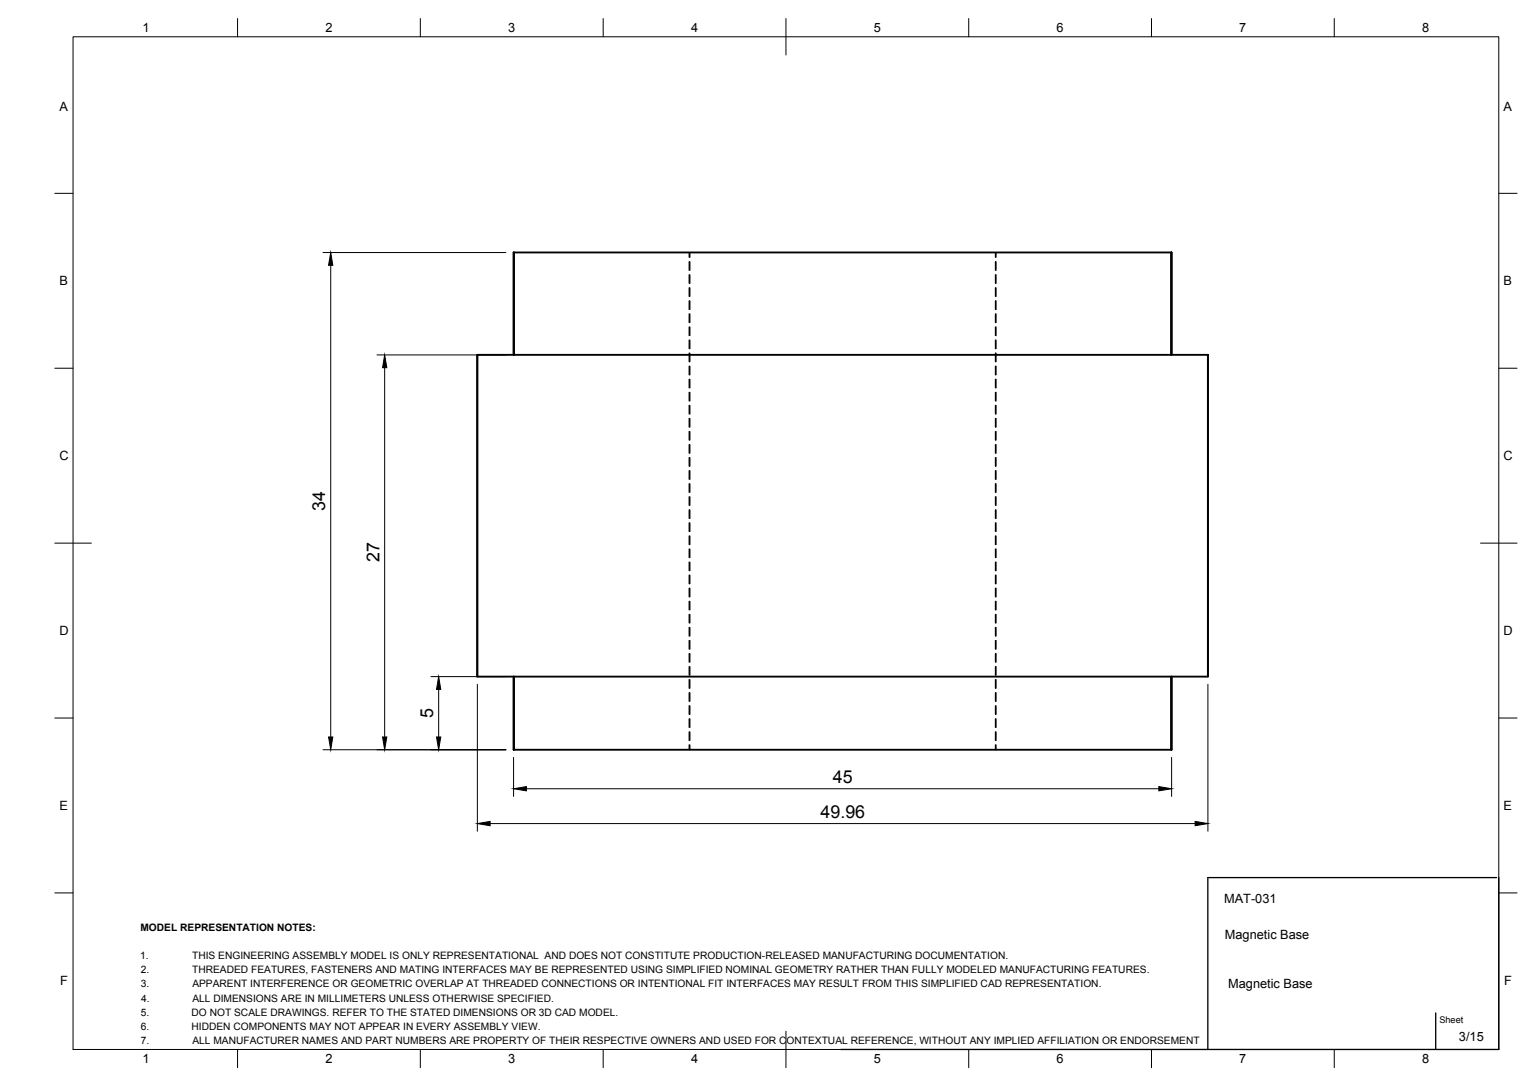
ISO-10303-21;
HEADER;
/* Generated by software containing ST-Developer
 * from STEP Tools, Inc. (www.steptools.com) 
 */

FILE_DESCRIPTION(
/* description */ ('STEP AP214'),
/* implementation_level */ '2;1');

FILE_NAME(
/* name */ 'Magnetic Base.step',
/* time_stamp */ '2026-11-14T06:58:01-08:00',
/* author */ (''),
/* organization */ (''),
/* preprocessor_version */ 'ST-DEVELOPER v20.2',
/* originating_system */ 'Autodesk Translation Framework v15.17.0.0',
/* authorisation */ '');

FILE_SCHEMA (('AUTOMOTIVE_DESIGN { 1 0 10303 214 3 1 1 }'));
ENDSEC;

DATA;
#10=MECHANICAL_DESIGN_GEOMETRIC_PRESENTATION_REPRESENTATION('',(#1140,#1141,#1142,#1143),#38635);
#1112=SHAPE_REPRESENTATION_RELATIONSHIP('SRR','None',#38685,#1126);
#1126=ADVANCED_BREP_SHAPE_REPRESENTATION('',(#1166,#1167,#1168,#1169),#38621);
#1140=STYLED_ITEM('',(#38764),#1166);
#1141=STYLED_ITEM('',(#38764),#1167);
#1142=STYLED_ITEM('',(#38764),#1168);
#1143=STYLED_ITEM('',(#38764),#1169);
#1166=MANIFOLD_SOLID_BREP('Body1',#17606);
#1167=MANIFOLD_SOLID_BREP('Body2',#17607);
#1168=MANIFOLD_SOLID_BREP('Body3',#17608);
#1169=MANIFOLD_SOLID_BREP('Body4',#17609);
#1192=PLANE('',#17795);
#1193=PLANE('',#17796);
#1194=PLANE('',#17797);
#1195=PLANE('',#17800);
#1196=PLANE('',#17803);
#1197=PLANE('',#17804);
#1198=PLANE('',#17816);
#1199=PLANE('',#17817);
#1200=PLANE('',#17818);
#1201=PLANE('',#17819);
#1202=PLANE('',#17821);
#1203=PLANE('',#17824);
#1204=PLANE('',#17825);
#1205=PLANE('',#17826);
#1206=PLANE('',#17827);
#1207=PLANE('',#17828);
#1208=PLANE('',#17831);
#1209=PLANE('',#17835);
#1210=PLANE('',#17838);
#1211=PLANE('',#17841);
#1212=PLANE('',#17842);
#1213=PLANE('',#17843);
#1214=PLANE('',#17844);
#1215=PLANE('',#17847);
#1216=PLANE('',#17851);
#1217=PLANE('',#17854);
#1641=FACE_OUTER_BOUND('',#2647,.T.);
#1642=FACE_OUTER_BOUND('',#2648,.T.);
#1643=FACE_OUTER_BOUND('',#2649,.T.);
#1644=FACE_OUTER_BOUND('',#2650,.T.);
#1645=FACE_OUTER_BOUND('',#2651,.T.);
#1646=FACE_OUTER_BOUND('',#2652,.T.);
#1647=FACE_OUTER_BOUND('',#2653,.T.);
#1648=FACE_OUTER_BOUND('',#2654,.T.);
#1649=FACE_OUTER_BOUND('',#2655,.T.);
#1650=FACE_OUTER_BOUND('',#2656,.T.);
#1651=FACE_OUTER_BOUND('',#2657,.T.);
#1652=FACE_OUTER_BOUND('',#2658,.T.);
#1653=FACE_OUTER_BOUND('',#2659,.T.);
#1654=FACE_OUTER_BOUND('',#2660,.T.);
#1655=FACE_OUTER_BOUND('',#2661,.T.);
#1656=FACE_OUTER_BOUND('',#2662,.T.);
#1657=FACE_OUTER_BOUND('',#2663,.T.);
#1658=FACE_OUTER_BOUND('',#2664,.T.);
#1659=FACE_OUTER_BOUND('',#2665,.T.);
#1660=FACE_OUTER_BOUND('',#2666,.T.);
#1661=FACE_OUTER_BOUND('',#2667,.T.);
#1662=FACE_OUTER_BOUND('',#2668,.T.);
#1663=FACE_OUTER_BOUND('',#2669,.T.);
#1664=FACE_OUTER_BOUND('',#2670,.T.);
#1665=FACE_OUTER_BOUND('',#2671,.T.);
#1666=FACE_OUTER_BOUND('',#2672,.T.);
#1667=FACE_OUTER_BOUND('',#2673,.T.);
#1668=FACE_OUTER_BOUND('',#2674,.T.);
#1669=FACE_OUTER_BOUND('',#2675,.T.);
#1670=FACE_OUTER_BOUND('',#2676,.T.);
#1671=FACE_OUTER_BOUND('',#2677,.T.);
#1672=FACE_OUTER_BOUND('',#2678,.T.);
#1673=FACE_OUTER_BOUND('',#2679,.T.);
#1674=FACE_OUTER_BOUND('',#2680,.T.);
#1675=FACE_OUTER_BOUND('',#2681,.T.);
#1676=FACE_OUTER_BOUND('',#2682,.T.);
#1677=FACE_OUTER_BOUND('',#2683,.T.);
#1678=FACE_OUTER_BOUND('',#2684,.T.);
#1679=FACE_OUTER_BOUND('',#2685,.T.);
#1680=FACE_OUTER_BOUND('',#2686,.T.);
#2647=EDGE_LOOP('',(#10909,#10910,#10911,#10912));
#2648=EDGE_LOOP('',(#10913,#10914,#10915,#10916));
#2649=EDGE_LOOP('',(#10917,#10918,#10919,#10920,#10921,#10922,#10923,#10924));
#2650=EDGE_LOOP('',(#10925,#10926,#10927,#10928,#10929,#10930,#10931,#10932));
#2651=EDGE_LOOP('',(#10933,#10934,#10935,#10936));
#2652=EDGE_LOOP('',(#10937,#10938,#10939,#10940));
#2653=EDGE_LOOP('',(#10941,#10942,#10943,#10944));
#2654=EDGE_LOOP('',(#10945,#10946,#10947,#10948));
#2655=EDGE_LOOP('',(#10949,#10950,#10951,#10952));
#2656=EDGE_LOOP('',(#10953,#10954,#10955,#10956));
#2657=EDGE_LOOP('',(#10957,#10958,#10959,#10960));
#2658=EDGE_LOOP('',(#10961,#10962,#10963,#10964));
#2659=EDGE_LOOP('',(#10965,#10966,#10967,#10968));
#2660=EDGE_LOOP('',(#10969,#10970,#10971,#10972,#10973,#10974,#10975,#10976));
#2661=EDGE_LOOP('',(#10977,#10978,#10979,#10980,#10981,#10982,#10983,#10984));
#2662=EDGE_LOOP('',(#10985,#10986,#10987,#10988));
#2663=EDGE_LOOP('',(#10989,#10990,#10991,#10992));
#2664=EDGE_LOOP('',(#10993,#10994,#10995,#10996));
#2665=EDGE_LOOP('',(#10997,#10998,#10999,#11000));
#2666=EDGE_LOOP('',(#11001,#11002,#11003,#11004));
#2667=EDGE_LOOP('',(#11005,#11006,#11007,#11008));
#2668=EDGE_LOOP('',(#11009,#11010,#11011,#11012,#11013,#11014,#11015,#11016));
#2669=EDGE_LOOP('',(#11017,#11018,#11019,#11020,#11021,#11022,#11023,#11024));
#2670=EDGE_LOOP('',(#11025,#11026,#11027,#11028));
#2671=EDGE_LOOP('',(#11029,#11030,#11031,#11032));
#2672=EDGE_LOOP('',(#11033,#11034,#11035,#11036));
#2673=EDGE_LOOP('',(#11037,#11038,#11039,#11040));
#2674=EDGE_LOOP('',(#11041,#11042,#11043,#11044));
#2675=EDGE_LOOP('',(#11045,#11046,#11047,#11048));
#2676=EDGE_LOOP('',(#11049,#11050,#11051,#11052));
#2677=EDGE_LOOP('',(#11053,#11054,#11055,#11056));
#2678=EDGE_LOOP('',(#11057,#11058,#11059,#11060,#11061,#11062,#11063,#11064));
#2679=EDGE_LOOP('',(#11065,#11066,#11067,#11068,#11069,#11070,#11071,#11072));
#2680=EDGE_LOOP('',(#11073,#11074,#11075,#11076));
#2681=EDGE_LOOP('',(#11077,#11078,#11079,#11080));
#2682=EDGE_LOOP('',(#11081,#11082,#11083,#11084));
#2683=EDGE_LOOP('',(#11085,#11086,#11087,#11088));
#2684=EDGE_LOOP('',(#11089,#11090,#11091,#11092));
#2685=EDGE_LOOP('',(#11093,#11094,#11095,#11096));
#2686=EDGE_LOOP('',(#11097,#11098,#11099,#11100));
#3698=LINE('',#24606,#4642);
#3699=LINE('',#24609,#4643);
#3700=LINE('',#24615,#4644);
#3701=LINE('',#24618,#4645);
#3702=LINE('',#24621,#4646);
#3703=LINE('',#24623,#4647);
#3704=LINE('',#24625,#4648);
#3705=LINE('',#24627,#4649);
#3706=LINE('',#24628,#4650);
#3707=LINE('',#24629,#4651);
#3708=LINE('',#24632,#4652);
#3709=LINE('',#24633,#4653);
#3710=LINE('',#24635,#4654);
#3711=LINE('',#24637,#4655);
#3712=LINE('',#24639,#4656);
#3713=LINE('',#24640,#4657);
#3714=LINE('',#24656,#4658);
#3715=LINE('',#24659,#4659);
#3716=LINE('',#24665,#4660);
#3717=LINE('',#24668,#4661);
#3718=LINE('',#24674,#4662);
#3719=LINE('',#24677,#4663);
#3720=LINE('',#24679,#4664);
#3721=LINE('',#24680,#4665);
#3722=LINE('',#24682,#4666);
#3723=LINE('',#24684,#4667);
#3724=LINE('',#24685,#4668);
#3725=LINE('',#24687,#4669);
#3726=LINE('',#24689,#4670);
#3727=LINE('',#24691,#4671);
#3728=LINE('',#24692,#4672);
#3729=LINE('',#24693,#4673);
#3730=LINE('',#24704,#4674);
#3731=LINE('',#24706,#4675);
#3732=LINE('',#24708,#4676);
#3733=LINE('',#24709,#4677);
#3734=LINE('',#24713,#4678);
#3735=LINE('',#24714,#4679);
#3736=LINE('',#24716,#4680);
#3737=LINE('',#24718,#4681);
#3738=LINE('',#24720,#4682);
#3739=LINE('',#24722,#4683);
#3740=LINE('',#24723,#4684);
#3741=LINE('',#24726,#4685);
#3742=LINE('',#24728,#4686);
#3743=LINE('',#24730,#4687);
#3744=LINE('',#24732,#4688);
#3745=LINE('',#24734,#4689);
#3746=LINE('',#24736,#4690);
#3747=LINE('',#24737,#4691);
#3748=LINE('',#24754,#4692);
#3749=LINE('',#24756,#4693);
#3750=LINE('',#24758,#4694);
#3751=LINE('',#24759,#4695);
#3752=LINE('',#24763,#4696);
#3753=LINE('',#24764,#4697);
#3754=LINE('',#24766,#4698);
#3755=LINE('',#24768,#4699);
#3756=LINE('',#24770,#4700);
#3757=LINE('',#24772,#4701);
#3758=LINE('',#24773,#4702);
#3759=LINE('',#24776,#4703);
#3760=LINE('',#24778,#4704);
#3761=LINE('',#24780,#4705);
#3762=LINE('',#24782,#4706);
#3763=LINE('',#24784,#4707);
#3764=LINE('',#24786,#4708);
#3765=LINE('',#24787,#4709);
#4642=VECTOR('',#19751,1000.);
#4643=VECTOR('',#19754,1000.);
#4644=VECTOR('',#19759,1000.);
#4645=VECTOR('',#19762,1000.);
#4646=VECTOR('',#19765,1000.);
#4647=VECTOR('',#19766,1000.);
#4648=VECTOR('',#19767,1000.);
#4649=VECTOR('',#19768,1000.);
#4650=VECTOR('',#19769,1000.);
#4651=VECTOR('',#19770,1000.);
#4652=VECTOR('',#19773,1000.);
#4653=VECTOR('',#19774,1000.);
#4654=VECTOR('',#19775,1000.);
#4655=VECTOR('',#19776,1000.);
#4656=VECTOR('',#19777,1000.);
#4657=VECTOR('',#19778,1000.);
#4658=VECTOR('',#19803,1000.);
#4659=VECTOR('',#19806,1000.);
#4660=VECTOR('',#19811,1000.);
#4661=VECTOR('',#19814,1000.);
#4662=VECTOR('',#19819,1000.);
#4663=VECTOR('',#19822,1000.);
#4664=VECTOR('',#19825,1000.);
#4665=VECTOR('',#19826,1000.);
#4666=VECTOR('',#19827,1000.);
#4667=VECTOR('',#19828,1000.);
#4668=VECTOR('',#19829,1000.);
#4669=VECTOR('',#19832,1000.);
#4670=VECTOR('',#19833,1000.);
#4671=VECTOR('',#19834,1000.);
#4672=VECTOR('',#19835,1000.);
#4673=VECTOR('',#19836,1000.);
#4674=VECTOR('',#19853,1000.);
#4675=VECTOR('',#19854,1000.);
#4676=VECTOR('',#19855,1000.);
#4677=VECTOR('',#19856,1000.);
#4678=VECTOR('',#19859,1000.);
#4679=VECTOR('',#19860,1000.);
#4680=VECTOR('',#19861,1000.);
#4681=VECTOR('',#19862,1000.);
#4682=VECTOR('',#19863,1000.);
#4683=VECTOR('',#19864,1000.);
#4684=VECTOR('',#19865,1000.);
#4685=VECTOR('',#19868,1000.);
#4686=VECTOR('',#19869,1000.);
#4687=VECTOR('',#19870,1000.);
#4688=VECTOR('',#19871,1000.);
#4689=VECTOR('',#19872,1000.);
#4690=VECTOR('',#19873,1000.);
#4691=VECTOR('',#19874,1000.);
#4692=VECTOR('',#19903,1000.);
#4693=VECTOR('',#19904,1000.);
#4694=VECTOR('',#19905,1000.);
#4695=VECTOR('',#19906,1000.);
#4696=VECTOR('',#19909,1000.);
#4697=VECTOR('',#19910,1000.);
#4698=VECTOR('',#19911,1000.);
#4699=VECTOR('',#19912,1000.);
#4700=VECTOR('',#19913,1000.);
#4701=VECTOR('',#19914,1000.);
#4702=VECTOR('',#19915,1000.);
#4703=VECTOR('',#19918,1000.);
#4704=VECTOR('',#19919,1000.);
#4705=VECTOR('',#19920,1000.);
#4706=VECTOR('',#19921,1000.);
#4707=VECTOR('',#19922,1000.);
#4708=VECTOR('',#19923,1000.);
#4709=VECTOR('',#19924,1000.);
#5586=CIRCLE('',#17790,22.5);
#5587=CIRCLE('',#17791,22.5);
#5588=CIRCLE('',#17793,25.);
#5589=CIRCLE('',#17794,25.);
#5590=CIRCLE('',#17798,22.5);
#5591=CIRCLE('',#17799,10.5);
#5592=CIRCLE('',#17801,10.5);
#5593=CIRCLE('',#17805,22.5);
#5594=CIRCLE('',#17808,22.5);
#5595=CIRCLE('',#17809,22.5);
#5596=CIRCLE('',#17811,10.5);
#5597=CIRCLE('',#17812,10.5);
#5598=CIRCLE('',#17814,25.);
#5599=CIRCLE('',#17815,25.);
#5600=CIRCLE('',#17820,22.5);
#5601=CIRCLE('',#17822,22.5);
#5602=CIRCLE('',#17829,22.5);
#5603=CIRCLE('',#17830,10.5);
#5604=CIRCLE('',#17832,22.5);
#5605=CIRCLE('',#17833,10.5);
#5606=CIRCLE('',#17836,22.5);
#5607=CIRCLE('',#17839,22.5);
#5608=CIRCLE('',#17845,22.5);
#5609=CIRCLE('',#17846,10.5);
#5610=CIRCLE('',#17848,22.5);
#5611=CIRCLE('',#17849,10.5);
#5612=CIRCLE('',#17852,22.5);
#5613=CIRCLE('',#17855,22.5);
#6512=VERTEX_POINT('',#24602);
#6513=VERTEX_POINT('',#24603);
#6514=VERTEX_POINT('',#24605);
#6515=VERTEX_POINT('',#24607);
#6516=VERTEX_POINT('',#24611);
#6517=VERTEX_POINT('',#24612);
#6518=VERTEX_POINT('',#24614);
#6519=VERTEX_POINT('',#24616);
#6520=VERTEX_POINT('',#24620);
#6521=VERTEX_POINT('',#24622);
#6522=VERTEX_POINT('',#24624);
#6523=VERTEX_POINT('',#24626);
#6524=VERTEX_POINT('',#24631);
#6525=VERTEX_POINT('',#24634);
#6526=VERTEX_POINT('',#24636);
#6527=VERTEX_POINT('',#24638);
#6528=VERTEX_POINT('',#24652);
#6529=VERTEX_POINT('',#24653);
#6530=VERTEX_POINT('',#24655);
#6531=VERTEX_POINT('',#24657);
#6532=VERTEX_POINT('',#24661);
#6533=VERTEX_POINT('',#24662);
#6534=VERTEX_POINT('',#24664);
#6535=VERTEX_POINT('',#24666);
#6536=VERTEX_POINT('',#24670);
#6537=VERTEX_POINT('',#24671);
#6538=VERTEX_POINT('',#24673);
#6539=VERTEX_POINT('',#24675);
#6540=VERTEX_POINT('',#24681);
#6541=VERTEX_POINT('',#24683);
#6542=VERTEX_POINT('',#24688);
#6543=VERTEX_POINT('',#24690);
#6544=VERTEX_POINT('',#24702);
#6545=VERTEX_POINT('',#24703);
#6546=VERTEX_POINT('',#24705);
#6547=VERTEX_POINT('',#24707);
#6548=VERTEX_POINT('',#24711);
#6549=VERTEX_POINT('',#24712);
#6550=VERTEX_POINT('',#24715);
#6551=VERTEX_POINT('',#24717);
#6552=VERTEX_POINT('',#24719);
#6553=VERTEX_POINT('',#24721);
#6554=VERTEX_POINT('',#24725);
#6555=VERTEX_POINT('',#24727);
#6556=VERTEX_POINT('',#24729);
#6557=VERTEX_POINT('',#24731);
#6558=VERTEX_POINT('',#24733);
#6559=VERTEX_POINT('',#24735);
#6560=VERTEX_POINT('',#24752);
#6561=VERTEX_POINT('',#24753);
#6562=VERTEX_POINT('',#24755);
#6563=VERTEX_POINT('',#24757);
#6564=VERTEX_POINT('',#24761);
#6565=VERTEX_POINT('',#24762);
#6566=VERTEX_POINT('',#24765);
#6567=VERTEX_POINT('',#24767);
#6568=VERTEX_POINT('',#24769);
#6569=VERTEX_POINT('',#24771);
#6570=VERTEX_POINT('',#24775);
#6571=VERTEX_POINT('',#24777);
#6572=VERTEX_POINT('',#24779);
#6573=VERTEX_POINT('',#24781);
#6574=VERTEX_POINT('',#24783);
#6575=VERTEX_POINT('',#24785);
#8241=EDGE_CURVE('',#6512,#6513,#5586,.T.);
#8242=EDGE_CURVE('',#6513,#6514,#3698,.T.);
#8243=EDGE_CURVE('',#6515,#6514,#5587,.T.);
#8244=EDGE_CURVE('',#6515,#6512,#3699,.T.);
#8245=EDGE_CURVE('',#6516,#6517,#5588,.T.);
#8246=EDGE_CURVE('',#6516,#6518,#3700,.T.);
#8247=EDGE_CURVE('',#6519,#6518,#5589,.T.);
#8248=EDGE_CURVE('',#6519,#6517,#3701,.T.);
#8249=EDGE_CURVE('',#6520,#6516,#3702,.T.);
#8250=EDGE_CURVE('',#6521,#6520,#3703,.T.);
#8251=EDGE_CURVE('',#6522,#6521,#3704,.T.);
#8252=EDGE_CURVE('',#6522,#6523,#3705,.T.);
#8253=EDGE_CURVE('',#6523,#6514,#3706,.T.);
#8254=EDGE_CURVE('',#6518,#6513,#3707,.T.);
#8255=EDGE_CURVE('',#6517,#6524,#3708,.T.);
#8256=EDGE_CURVE('',#6512,#6519,#3709,.T.);
#8257=EDGE_CURVE('',#6515,#6525,#3710,.T.);
#8258=EDGE_CURVE('',#6525,#6526,#3711,.T.);
#8259=EDGE_CURVE('',#6527,#6526,#3712,.T.);
#8260=EDGE_CURVE('',#6524,#6527,#3713,.T.);
#8261=EDGE_CURVE('',#6521,#6527,#5590,.T.);
#8262=EDGE_CURVE('',#6526,#6522,#5591,.T.);
#8263=EDGE_CURVE('',#6525,#6523,#5592,.T.);
#8264=EDGE_CURVE('',#6520,#6524,#5593,.T.);
#8265=EDGE_CURVE('',#6528,#6529,#5594,.T.);
#8266=EDGE_CURVE('',#6529,#6530,#3714,.T.);
#8267=EDGE_CURVE('',#6530,#6531,#5595,.T.);
#8268=EDGE_CURVE('',#6531,#6528,#3715,.T.);
#8269=EDGE_CURVE('',#6532,#6533,#5596,.T.);
#8270=EDGE_CURVE('',#6534,#6533,#3716,.T.);
#8271=EDGE_CURVE('',#6535,#6534,#5597,.T.);
#8272=EDGE_CURVE('',#6532,#6535,#3717,.T.);
#8273=EDGE_CURVE('',#6536,#6537,#5598,.T.);
#8274=EDGE_CURVE('',#6536,#6538,#3718,.T.);
#8275=EDGE_CURVE('',#6539,#6538,#5599,.T.);
#8276=EDGE_CURVE('',#6539,#6537,#3719,.T.);
#8277=EDGE_CURVE('',#6528,#6539,#3720,.T.);
#8278=EDGE_CURVE('',#6534,#6531,#3721,.T.);
#8279=EDGE_CURVE('',#6533,#6540,#3722,.T.);
#8280=EDGE_CURVE('',#6541,#6540,#3723,.T.);
#8281=EDGE_CURVE('',#6537,#6541,#3724,.T.);
#8282=EDGE_CURVE('',#6538,#6529,#3725,.T.);
#8283=EDGE_CURVE('',#6542,#6536,#3726,.T.);
#8284=EDGE_CURVE('',#6543,#6542,#3727,.T.);
#8285=EDGE_CURVE('',#6543,#6532,#3728,.T.);
#8286=EDGE_CURVE('',#6530,#6535,#3729,.T.);
#8287=EDGE_CURVE('',#6543,#6540,#5600,.T.);
#8288=EDGE_CURVE('',#6542,#6541,#5601,.T.);
#8289=EDGE_CURVE('',#6544,#6545,#3730,.T.);
#8290=EDGE_CURVE('',#6544,#6546,#3731,.T.);
#8291=EDGE_CURVE('',#6546,#6547,#3732,.T.);
#8292=EDGE_CURVE('',#6547,#6545,#3733,.T.);
#8293=EDGE_CURVE('',#6548,#6549,#3734,.T.);
#8294=EDGE_CURVE('',#6549,#6544,#3735,.T.);
#8295=EDGE_CURVE('',#6545,#6550,#3736,.T.);
#8296=EDGE_CURVE('',#6550,#6551,#3737,.T.);
#8297=EDGE_CURVE('',#6552,#6551,#3738,.T.);
#8298=EDGE_CURVE('',#6553,#6552,#3739,.T.);
#8299=EDGE_CURVE('',#6553,#6548,#3740,.T.);
#8300=EDGE_CURVE('',#6546,#6554,#3741,.T.);
#8301=EDGE_CURVE('',#6554,#6555,#3742,.T.);
#8302=EDGE_CURVE('',#6555,#6556,#3743,.T.);
#8303=EDGE_CURVE('',#6556,#6557,#3744,.T.);
#8304=EDGE_CURVE('',#6558,#6557,#3745,.T.);
#8305=EDGE_CURVE('',#6558,#6559,#3746,.T.);
#8306=EDGE_CURVE('',#6559,#6547,#3747,.T.);
#8307=EDGE_CURVE('',#6555,#6548,#5602,.T.);
#8308=EDGE_CURVE('',#6556,#6553,#5603,.T.);
#8309=EDGE_CURVE('',#6551,#6558,#5604,.T.);
#8310=EDGE_CURVE('',#6557,#6552,#5605,.T.);
#8311=EDGE_CURVE('',#6550,#6559,#5606,.T.);
#8312=EDGE_CURVE('',#6554,#6549,#5607,.T.);
#8313=EDGE_CURVE('',#6560,#6561,#3748,.T.);
#8314=EDGE_CURVE('',#6560,#6562,#3749,.T.);
#8315=EDGE_CURVE('',#6562,#6563,#3750,.T.);
#8316=EDGE_CURVE('',#6563,#6561,#3751,.T.);
#8317=EDGE_CURVE('',#6564,#6565,#3752,.T.);
#8318=EDGE_CURVE('',#6565,#6560,#3753,.T.);
#8319=EDGE_CURVE('',#6561,#6566,#3754,.T.);
#8320=EDGE_CURVE('',#6566,#6567,#3755,.T.);
#8321=EDGE_CURVE('',#6568,#6567,#3756,.T.);
#8322=EDGE_CURVE('',#6569,#6568,#3757,.T.);
#8323=EDGE_CURVE('',#6569,#6564,#3758,.T.);
#8324=EDGE_CURVE('',#6562,#6570,#3759,.T.);
#8325=EDGE_CURVE('',#6570,#6571,#3760,.T.);
#8326=EDGE_CURVE('',#6571,#6572,#3761,.T.);
#8327=EDGE_CURVE('',#6572,#6573,#3762,.T.);
#8328=EDGE_CURVE('',#6574,#6573,#3763,.T.);
#8329=EDGE_CURVE('',#6574,#6575,#3764,.T.);
#8330=EDGE_CURVE('',#6575,#6563,#3765,.T.);
#8331=EDGE_CURVE('',#6571,#6564,#5608,.T.);
#8332=EDGE_CURVE('',#6572,#6569,#5609,.T.);
#8333=EDGE_CURVE('',#6567,#6574,#5610,.T.);
#8334=EDGE_CURVE('',#6573,#6568,#5611,.T.);
#8335=EDGE_CURVE('',#6566,#6575,#5612,.T.);
#8336=EDGE_CURVE('',#6570,#6565,#5613,.T.);
#10909=ORIENTED_EDGE('',*,*,#8241,.T.);
#10910=ORIENTED_EDGE('',*,*,#8242,.T.);
#10911=ORIENTED_EDGE('',*,*,#8243,.F.);
#10912=ORIENTED_EDGE('',*,*,#8244,.T.);
#10913=ORIENTED_EDGE('',*,*,#8245,.F.);
#10914=ORIENTED_EDGE('',*,*,#8246,.T.);
#10915=ORIENTED_EDGE('',*,*,#8247,.F.);
#10916=ORIENTED_EDGE('',*,*,#8248,.T.);
#10917=ORIENTED_EDGE('',*,*,#8249,.F.);
#10918=ORIENTED_EDGE('',*,*,#8250,.F.);
#10919=ORIENTED_EDGE('',*,*,#8251,.F.);
#10920=ORIENTED_EDGE('',*,*,#8252,.T.);
#10921=ORIENTED_EDGE('',*,*,#8253,.T.);
#10922=ORIENTED_EDGE('',*,*,#8242,.F.);
#10923=ORIENTED_EDGE('',*,*,#8254,.F.);
#10924=ORIENTED_EDGE('',*,*,#8246,.F.);
#10925=ORIENTED_EDGE('',*,*,#8255,.F.);
#10926=ORIENTED_EDGE('',*,*,#8248,.F.);
#10927=ORIENTED_EDGE('',*,*,#8256,.F.);
#10928=ORIENTED_EDGE('',*,*,#8244,.F.);
#10929=ORIENTED_EDGE('',*,*,#8257,.T.);
#10930=ORIENTED_EDGE('',*,*,#8258,.T.);
#10931=ORIENTED_EDGE('',*,*,#8259,.F.);
#10932=ORIENTED_EDGE('',*,*,#8260,.F.);
#10933=ORIENTED_EDGE('',*,*,#8261,.T.);
#10934=ORIENTED_EDGE('',*,*,#8259,.T.);
#10935=ORIENTED_EDGE('',*,*,#8262,.T.);
#10936=ORIENTED_EDGE('',*,*,#8251,.T.);
#10937=ORIENTED_EDGE('',*,*,#8257,.F.);
#10938=ORIENTED_EDGE('',*,*,#8243,.T.);
#10939=ORIENTED_EDGE('',*,*,#8253,.F.);
#10940=ORIENTED_EDGE('',*,*,#8263,.F.);
#10941=ORIENTED_EDGE('',*,*,#8258,.F.);
#10942=ORIENTED_EDGE('',*,*,#8263,.T.);
#10943=ORIENTED_EDGE('',*,*,#8252,.F.);
#10944=ORIENTED_EDGE('',*,*,#8262,.F.);
#10945=ORIENTED_EDGE('',*,*,#8254,.T.);
#10946=ORIENTED_EDGE('',*,*,#8241,.F.);
#10947=ORIENTED_EDGE('',*,*,#8256,.T.);
#10948=ORIENTED_EDGE('',*,*,#8247,.T.);
#10949=ORIENTED_EDGE('',*,*,#8249,.T.);
#10950=ORIENTED_EDGE('',*,*,#8245,.T.);
#10951=ORIENTED_EDGE('',*,*,#8255,.T.);
#10952=ORIENTED_EDGE('',*,*,#8264,.F.);
#10953=ORIENTED_EDGE('',*,*,#8250,.T.);
#10954=ORIENTED_EDGE('',*,*,#8264,.T.);
#10955=ORIENTED_EDGE('',*,*,#8260,.T.);
#10956=ORIENTED_EDGE('',*,*,#8261,.F.);
#10957=ORIENTED_EDGE('',*,*,#8265,.T.);
#10958=ORIENTED_EDGE('',*,*,#8266,.T.);
#10959=ORIENTED_EDGE('',*,*,#8267,.T.);
#10960=ORIENTED_EDGE('',*,*,#8268,.T.);
#10961=ORIENTED_EDGE('',*,*,#8269,.T.);
#10962=ORIENTED_EDGE('',*,*,#8270,.F.);
#10963=ORIENTED_EDGE('',*,*,#8271,.F.);
#10964=ORIENTED_EDGE('',*,*,#8272,.F.);
#10965=ORIENTED_EDGE('',*,*,#8273,.F.);
#10966=ORIENTED_EDGE('',*,*,#8274,.T.);
#10967=ORIENTED_EDGE('',*,*,#8275,.F.);
#10968=ORIENTED_EDGE('',*,*,#8276,.T.);
#10969=ORIENTED_EDGE('',*,*,#8277,.F.);
#10970=ORIENTED_EDGE('',*,*,#8268,.F.);
#10971=ORIENTED_EDGE('',*,*,#8278,.F.);
#10972=ORIENTED_EDGE('',*,*,#8270,.T.);
#10973=ORIENTED_EDGE('',*,*,#8279,.T.);
#10974=ORIENTED_EDGE('',*,*,#8280,.F.);
#10975=ORIENTED_EDGE('',*,*,#8281,.F.);
#10976=ORIENTED_EDGE('',*,*,#8276,.F.);
#10977=ORIENTED_EDGE('',*,*,#8282,.F.);
#10978=ORIENTED_EDGE('',*,*,#8274,.F.);
#10979=ORIENTED_EDGE('',*,*,#8283,.F.);
#10980=ORIENTED_EDGE('',*,*,#8284,.F.);
#10981=ORIENTED_EDGE('',*,*,#8285,.T.);
#10982=ORIENTED_EDGE('',*,*,#8272,.T.);
#10983=ORIENTED_EDGE('',*,*,#8286,.F.);
#10984=ORIENTED_EDGE('',*,*,#8266,.F.);
#10985=ORIENTED_EDGE('',*,*,#8267,.F.);
#10986=ORIENTED_EDGE('',*,*,#8286,.T.);
#10987=ORIENTED_EDGE('',*,*,#8271,.T.);
#10988=ORIENTED_EDGE('',*,*,#8278,.T.);
#10989=ORIENTED_EDGE('',*,*,#8285,.F.);
#10990=ORIENTED_EDGE('',*,*,#8287,.T.);
#10991=ORIENTED_EDGE('',*,*,#8279,.F.);
#10992=ORIENTED_EDGE('',*,*,#8269,.F.);
#10993=ORIENTED_EDGE('',*,*,#8281,.T.);
#10994=ORIENTED_EDGE('',*,*,#8288,.F.);
#10995=ORIENTED_EDGE('',*,*,#8283,.T.);
#10996=ORIENTED_EDGE('',*,*,#8273,.T.);
#10997=ORIENTED_EDGE('',*,*,#8280,.T.);
#10998=ORIENTED_EDGE('',*,*,#8287,.F.);
#10999=ORIENTED_EDGE('',*,*,#8284,.T.);
#11000=ORIENTED_EDGE('',*,*,#8288,.T.);
#11001=ORIENTED_EDGE('',*,*,#8277,.T.);
#11002=ORIENTED_EDGE('',*,*,#8275,.T.);
#11003=ORIENTED_EDGE('',*,*,#8282,.T.);
#11004=ORIENTED_EDGE('',*,*,#8265,.F.);
#11005=ORIENTED_EDGE('',*,*,#8289,.F.);
#11006=ORIENTED_EDGE('',*,*,#8290,.T.);
#11007=ORIENTED_EDGE('',*,*,#8291,.T.);
#11008=ORIENTED_EDGE('',*,*,#8292,.T.);
#11009=ORIENTED_EDGE('',*,*,#8293,.T.);
#11010=ORIENTED_EDGE('',*,*,#8294,.T.);
#11011=ORIENTED_EDGE('',*,*,#8289,.T.);
#11012=ORIENTED_EDGE('',*,*,#8295,.T.);
#11013=ORIENTED_EDGE('',*,*,#8296,.T.);
#11014=ORIENTED_EDGE('',*,*,#8297,.F.);
#11015=ORIENTED_EDGE('',*,*,#8298,.F.);
#11016=ORIENTED_EDGE('',*,*,#8299,.T.);
#11017=ORIENTED_EDGE('',*,*,#8291,.F.);
#11018=ORIENTED_EDGE('',*,*,#8300,.T.);
#11019=ORIENTED_EDGE('',*,*,#8301,.T.);
#11020=ORIENTED_EDGE('',*,*,#8302,.T.);
#11021=ORIENTED_EDGE('',*,*,#8303,.T.);
#11022=ORIENTED_EDGE('',*,*,#8304,.F.);
#11023=ORIENTED_EDGE('',*,*,#8305,.T.);
#11024=ORIENTED_EDGE('',*,*,#8306,.T.);
#11025=ORIENTED_EDGE('',*,*,#8307,.T.);
#11026=ORIENTED_EDGE('',*,*,#8299,.F.);
#11027=ORIENTED_EDGE('',*,*,#8308,.F.);
#11028=ORIENTED_EDGE('',*,*,#8302,.F.);
#11029=ORIENTED_EDGE('',*,*,#8297,.T.);
#11030=ORIENTED_EDGE('',*,*,#8309,.T.);
#11031=ORIENTED_EDGE('',*,*,#8304,.T.);
#11032=ORIENTED_EDGE('',*,*,#8310,.T.);
#11033=ORIENTED_EDGE('',*,*,#8310,.F.);
#11034=ORIENTED_EDGE('',*,*,#8303,.F.);
#11035=ORIENTED_EDGE('',*,*,#8308,.T.);
#11036=ORIENTED_EDGE('',*,*,#8298,.T.);
#11037=ORIENTED_EDGE('',*,*,#8292,.F.);
#11038=ORIENTED_EDGE('',*,*,#8306,.F.);
#11039=ORIENTED_EDGE('',*,*,#8311,.F.);
#11040=ORIENTED_EDGE('',*,*,#8295,.F.);
#11041=ORIENTED_EDGE('',*,*,#8311,.T.);
#11042=ORIENTED_EDGE('',*,*,#8305,.F.);
#11043=ORIENTED_EDGE('',*,*,#8309,.F.);
#11044=ORIENTED_EDGE('',*,*,#8296,.F.);
#11045=ORIENTED_EDGE('',*,*,#8312,.F.);
#11046=ORIENTED_EDGE('',*,*,#8300,.F.);
#11047=ORIENTED_EDGE('',*,*,#8290,.F.);
#11048=ORIENTED_EDGE('',*,*,#8294,.F.);
#11049=ORIENTED_EDGE('',*,*,#8307,.F.);
#11050=ORIENTED_EDGE('',*,*,#8301,.F.);
#11051=ORIENTED_EDGE('',*,*,#8312,.T.);
#11052=ORIENTED_EDGE('',*,*,#8293,.F.);
#11053=ORIENTED_EDGE('',*,*,#8313,.F.);
#11054=ORIENTED_EDGE('',*,*,#8314,.T.);
#11055=ORIENTED_EDGE('',*,*,#8315,.T.);
#11056=ORIENTED_EDGE('',*,*,#8316,.T.);
#11057=ORIENTED_EDGE('',*,*,#8317,.T.);
#11058=ORIENTED_EDGE('',*,*,#8318,.T.);
#11059=ORIENTED_EDGE('',*,*,#8313,.T.);
#11060=ORIENTED_EDGE('',*,*,#8319,.T.);
#11061=ORIENTED_EDGE('',*,*,#8320,.T.);
#11062=ORIENTED_EDGE('',*,*,#8321,.F.);
#11063=ORIENTED_EDGE('',*,*,#8322,.F.);
#11064=ORIENTED_EDGE('',*,*,#8323,.T.);
#11065=ORIENTED_EDGE('',*,*,#8315,.F.);
#11066=ORIENTED_EDGE('',*,*,#8324,.T.);
#11067=ORIENTED_EDGE('',*,*,#8325,.T.);
#11068=ORIENTED_EDGE('',*,*,#8326,.T.);
#11069=ORIENTED_EDGE('',*,*,#8327,.T.);
#11070=ORIENTED_EDGE('',*,*,#8328,.F.);
#11071=ORIENTED_EDGE('',*,*,#8329,.T.);
#11072=ORIENTED_EDGE('',*,*,#8330,.T.);
#11073=ORIENTED_EDGE('',*,*,#8331,.T.);
#11074=ORIENTED_EDGE('',*,*,#8323,.F.);
#11075=ORIENTED_EDGE('',*,*,#8332,.F.);
#11076=ORIENTED_EDGE('',*,*,#8326,.F.);
#11077=ORIENTED_EDGE('',*,*,#8321,.T.);
#11078=ORIENTED_EDGE('',*,*,#8333,.T.);
#11079=ORIENTED_EDGE('',*,*,#8328,.T.);
#11080=ORIENTED_EDGE('',*,*,#8334,.T.);
#11081=ORIENTED_EDGE('',*,*,#8334,.F.);
#11082=ORIENTED_EDGE('',*,*,#8327,.F.);
#11083=ORIENTED_EDGE('',*,*,#8332,.T.);
#11084=ORIENTED_EDGE('',*,*,#8322,.T.);
#11085=ORIENTED_EDGE('',*,*,#8316,.F.);
#11086=ORIENTED_EDGE('',*,*,#8330,.F.);
#11087=ORIENTED_EDGE('',*,*,#8335,.F.);
#11088=ORIENTED_EDGE('',*,*,#8319,.F.);
#11089=ORIENTED_EDGE('',*,*,#8335,.T.);
#11090=ORIENTED_EDGE('',*,*,#8329,.F.);
#11091=ORIENTED_EDGE('',*,*,#8333,.F.);
#11092=ORIENTED_EDGE('',*,*,#8320,.F.);
#11093=ORIENTED_EDGE('',*,*,#8336,.F.);
#11094=ORIENTED_EDGE('',*,*,#8324,.F.);
#11095=ORIENTED_EDGE('',*,*,#8314,.F.);
#11096=ORIENTED_EDGE('',*,*,#8318,.F.);
#11097=ORIENTED_EDGE('',*,*,#8331,.F.);
#11098=ORIENTED_EDGE('',*,*,#8325,.F.);
#11099=ORIENTED_EDGE('',*,*,#8336,.T.);
#11100=ORIENTED_EDGE('',*,*,#8317,.F.);
#16245=CYLINDRICAL_SURFACE('',#17789,22.5);
#16246=CYLINDRICAL_SURFACE('',#17792,25.);
#16247=CYLINDRICAL_SURFACE('',#17802,10.5);
#16248=CYLINDRICAL_SURFACE('',#17806,22.5);
#16249=CYLINDRICAL_SURFACE('',#17807,22.5);
#16250=CYLINDRICAL_SURFACE('',#17810,10.5);
#16251=CYLINDRICAL_SURFACE('',#17813,25.);
#16252=CYLINDRICAL_SURFACE('',#17823,22.5);
#16253=CYLINDRICAL_SURFACE('',#17834,10.5);
#16254=CYLINDRICAL_SURFACE('',#17837,22.5);
#16255=CYLINDRICAL_SURFACE('',#17840,22.5);
#16256=CYLINDRICAL_SURFACE('',#17850,10.5);
#16257=CYLINDRICAL_SURFACE('',#17853,22.5);
#16258=CYLINDRICAL_SURFACE('',#17856,22.5);
#16600=ADVANCED_FACE('',(#1641),#16245,.T.);
#16601=ADVANCED_FACE('',(#1642),#16246,.T.);
#16602=ADVANCED_FACE('',(#1643),#1192,.F.);
#16603=ADVANCED_FACE('',(#1644),#1193,.F.);
#16604=ADVANCED_FACE('',(#1645),#1194,.F.);
#16605=ADVANCED_FACE('',(#1646),#1195,.T.);
#16606=ADVANCED_FACE('',(#1647),#16247,.F.);
#16607=ADVANCED_FACE('',(#1648),#1196,.T.);
#16608=ADVANCED_FACE('',(#1649),#1197,.T.);
#16609=ADVANCED_FACE('',(#1650),#16248,.T.);
#16610=ADVANCED_FACE('',(#1651),#16249,.T.);
#16611=ADVANCED_FACE('',(#1652),#16250,.F.);
#16612=ADVANCED_FACE('',(#1653),#16251,.T.);
#16613=ADVANCED_FACE('',(#1654),#1198,.F.);
#16614=ADVANCED_FACE('',(#1655),#1199,.F.);
#16615=ADVANCED_FACE('',(#1656),#1200,.F.);
#16616=ADVANCED_FACE('',(#1657),#1201,.T.);
#16617=ADVANCED_FACE('',(#1658),#1202,.T.);
#16618=ADVANCED_FACE('',(#1659),#16252,.T.);
#16619=ADVANCED_FACE('',(#1660),#1203,.T.);
#16620=ADVANCED_FACE('',(#1661),#1204,.T.);
#16621=ADVANCED_FACE('',(#1662),#1205,.T.);
#16622=ADVANCED_FACE('',(#1663),#1206,.T.);
#16623=ADVANCED_FACE('',(#1664),#1207,.F.);
#16624=ADVANCED_FACE('',(#1665),#1208,.T.);
#16625=ADVANCED_FACE('',(#1666),#16253,.F.);
#16626=ADVANCED_FACE('',(#1667),#1209,.T.);
#16627=ADVANCED_FACE('',(#1668),#16254,.T.);
#16628=ADVANCED_FACE('',(#1669),#1210,.T.);
#16629=ADVANCED_FACE('',(#1670),#16255,.T.);
#16630=ADVANCED_FACE('',(#1671),#1211,.T.);
#16631=ADVANCED_FACE('',(#1672),#1212,.T.);
#16632=ADVANCED_FACE('',(#1673),#1213,.T.);
#16633=ADVANCED_FACE('',(#1674),#1214,.F.);
#16634=ADVANCED_FACE('',(#1675),#1215,.T.);
#16635=ADVANCED_FACE('',(#1676),#16256,.F.);
#16636=ADVANCED_FACE('',(#1677),#1216,.T.);
#16637=ADVANCED_FACE('',(#1678),#16257,.T.);
#16638=ADVANCED_FACE('',(#1679),#1217,.T.);
#16639=ADVANCED_FACE('',(#1680),#16258,.T.);
#17606=CLOSED_SHELL('',(#16600,#16601,#16602,#16603,#16604,#16605,#16606,
#16607,#16608,#16609));
#17607=CLOSED_SHELL('',(#16610,#16611,#16612,#16613,#16614,#16615,#16616,
#16617,#16618,#16619));
#17608=CLOSED_SHELL('',(#16620,#16621,#16622,#16623,#16624,#16625,#16626,
#16627,#16628,#16629));
#17609=CLOSED_SHELL('',(#16630,#16631,#16632,#16633,#16634,#16635,#16636,
#16637,#16638,#16639));
#17788=AXIS2_PLACEMENT_3D('',#24600,#19745,#19746);
#17789=AXIS2_PLACEMENT_3D('',#24601,#19747,#19748);
#17790=AXIS2_PLACEMENT_3D('',#24604,#19749,#19750);
#17791=AXIS2_PLACEMENT_3D('',#24608,#19752,#19753);
#17792=AXIS2_PLACEMENT_3D('',#24610,#19755,#19756);
#17793=AXIS2_PLACEMENT_3D('',#24613,#19757,#19758);
#17794=AXIS2_PLACEMENT_3D('',#24617,#19760,#19761);
#17795=AXIS2_PLACEMENT_3D('',#24619,#19763,#19764);
#17796=AXIS2_PLACEMENT_3D('',#24630,#19771,#19772);
#17797=AXIS2_PLACEMENT_3D('',#24641,#19779,#19780);
#17798=AXIS2_PLACEMENT_3D('',#24642,#19781,#19782);
#17799=AXIS2_PLACEMENT_3D('',#24643,#19783,#19784);
#17800=AXIS2_PLACEMENT_3D('',#24644,#19785,#19786);
#17801=AXIS2_PLACEMENT_3D('',#24645,#19787,#19788);
#17802=AXIS2_PLACEMENT_3D('',#24646,#19789,#19790);
#17803=AXIS2_PLACEMENT_3D('',#24647,#19791,#19792);
#17804=AXIS2_PLACEMENT_3D('',#24648,#19793,#19794);
#17805=AXIS2_PLACEMENT_3D('',#24649,#19795,#19796);
#17806=AXIS2_PLACEMENT_3D('',#24650,#19797,#19798);
#17807=AXIS2_PLACEMENT_3D('',#24651,#19799,#19800);
#17808=AXIS2_PLACEMENT_3D('',#24654,#19801,#19802);
#17809=AXIS2_PLACEMENT_3D('',#24658,#19804,#19805);
#17810=AXIS2_PLACEMENT_3D('',#24660,#19807,#19808);
#17811=AXIS2_PLACEMENT_3D('',#24663,#19809,#19810);
#17812=AXIS2_PLACEMENT_3D('',#24667,#19812,#19813);
#17813=AXIS2_PLACEMENT_3D('',#24669,#19815,#19816);
#17814=AXIS2_PLACEMENT_3D('',#24672,#19817,#19818);
#17815=AXIS2_PLACEMENT_3D('',#24676,#19820,#19821);
#17816=AXIS2_PLACEMENT_3D('',#24678,#19823,#19824);
#17817=AXIS2_PLACEMENT_3D('',#24686,#19830,#19831);
#17818=AXIS2_PLACEMENT_3D('',#24694,#19837,#19838);
#17819=AXIS2_PLACEMENT_3D('',#24695,#19839,#19840);
#17820=AXIS2_PLACEMENT_3D('',#24696,#19841,#19842);
#17821=AXIS2_PLACEMENT_3D('',#24697,#19843,#19844);
#17822=AXIS2_PLACEMENT_3D('',#24698,#19845,#19846);
#17823=AXIS2_PLACEMENT_3D('',#24699,#19847,#19848);
#17824=AXIS2_PLACEMENT_3D('',#24700,#19849,#19850);
#17825=AXIS2_PLACEMENT_3D('',#24701,#19851,#19852);
#17826=AXIS2_PLACEMENT_3D('',#24710,#19857,#19858);
#17827=AXIS2_PLACEMENT_3D('',#24724,#19866,#19867);
#17828=AXIS2_PLACEMENT_3D('',#24738,#19875,#19876);
#17829=AXIS2_PLACEMENT_3D('',#24739,#19877,#19878);
#17830=AXIS2_PLACEMENT_3D('',#24740,#19879,#19880);
#17831=AXIS2_PLACEMENT_3D('',#24741,#19881,#19882);
#17832=AXIS2_PLACEMENT_3D('',#24742,#19883,#19884);
#17833=AXIS2_PLACEMENT_3D('',#24743,#19885,#19886);
#17834=AXIS2_PLACEMENT_3D('',#24744,#19887,#19888);
#17835=AXIS2_PLACEMENT_3D('',#24745,#19889,#19890);
#17836=AXIS2_PLACEMENT_3D('',#24746,#19891,#19892);
#17837=AXIS2_PLACEMENT_3D('',#24747,#19893,#19894);
#17838=AXIS2_PLACEMENT_3D('',#24748,#19895,#19896);
#17839=AXIS2_PLACEMENT_3D('',#24749,#19897,#19898);
#17840=AXIS2_PLACEMENT_3D('',#24750,#19899,#19900);
#17841=AXIS2_PLACEMENT_3D('',#24751,#19901,#19902);
#17842=AXIS2_PLACEMENT_3D('',#24760,#19907,#19908);
#17843=AXIS2_PLACEMENT_3D('',#24774,#19916,#19917);
#17844=AXIS2_PLACEMENT_3D('',#24788,#19925,#19926);
#17845=AXIS2_PLACEMENT_3D('',#24789,#19927,#19928);
#17846=AXIS2_PLACEMENT_3D('',#24790,#19929,#19930);
#17847=AXIS2_PLACEMENT_3D('',#24791,#19931,#19932);
#17848=AXIS2_PLACEMENT_3D('',#24792,#19933,#19934);
#17849=AXIS2_PLACEMENT_3D('',#24793,#19935,#19936);
#17850=AXIS2_PLACEMENT_3D('',#24794,#19937,#19938);
#17851=AXIS2_PLACEMENT_3D('',#24795,#19939,#19940);
#17852=AXIS2_PLACEMENT_3D('',#24796,#19941,#19942);
#17853=AXIS2_PLACEMENT_3D('',#24797,#19943,#19944);
#17854=AXIS2_PLACEMENT_3D('',#24798,#19945,#19946);
#17855=AXIS2_PLACEMENT_3D('',#24799,#19947,#19948);
#17856=AXIS2_PLACEMENT_3D('',#24800,#19949,#19950);
#19745=DIRECTION('axis',(0.,0.,1.));
#19746=DIRECTION('refdir',(1.,0.,0.));
#19747=DIRECTION('center_axis',(0.,1.,0.));
#19748=DIRECTION('ref_axis',(0.,0.,1.));
#19749=DIRECTION('center_axis',(0.,1.,0.));
#19750=DIRECTION('ref_axis',(0.,0.,1.));
#19751=DIRECTION('',(0.,1.,0.));
#19752=DIRECTION('center_axis',(0.,1.,0.));
#19753=DIRECTION('ref_axis',(0.,0.,1.));
#19754=DIRECTION('',(0.,-1.,0.));
#19755=DIRECTION('center_axis',(0.,-1.,0.));
#19756=DIRECTION('ref_axis',(1.22464679914735E-16,0.,1.));
#19757=DIRECTION('center_axis',(0.,-1.,0.));
#19758=DIRECTION('ref_axis',(0.,0.,-1.));
#19759=DIRECTION('',(0.,1.,0.));
#19760=DIRECTION('center_axis',(0.,1.,0.));
#19761=DIRECTION('ref_axis',(0.,0.,1.));
#19762=DIRECTION('',(0.,-1.,0.));
#19763=DIRECTION('center_axis',(0.,0.,1.));
#19764=DIRECTION('ref_axis',(1.,0.,0.));
#19765=DIRECTION('',(1.,0.,0.));
#19766=DIRECTION('',(0.,1.,0.));
#19767=DIRECTION('',(1.,0.,0.));
#19768=DIRECTION('',(0.,1.,0.));
#19769=DIRECTION('',(1.,0.,0.));
#19770=DIRECTION('',(-1.,0.,0.));
#19771=DIRECTION('center_axis',(0.,0.,1.));
#19772=DIRECTION('ref_axis',(1.,0.,0.));
#19773=DIRECTION('',(1.,0.,0.));
#19774=DIRECTION('',(-1.,0.,0.));
#19775=DIRECTION('',(1.,0.,0.));
#19776=DIRECTION('',(0.,-1.,0.));
#19777=DIRECTION('',(1.,0.,0.));
#19778=DIRECTION('',(0.,-1.,0.));
#19779=DIRECTION('center_axis',(0.,1.,0.));
#19780=DIRECTION('ref_axis',(0.,0.,1.));
#19781=DIRECTION('center_axis',(0.,-1.,0.));
#19782=DIRECTION('ref_axis',(0.,0.,-1.));
#19783=DIRECTION('center_axis',(0.,1.,0.));
#19784=DIRECTION('ref_axis',(0.,0.,1.));
#19785=DIRECTION('center_axis',(0.,1.,0.));
#19786=DIRECTION('ref_axis',(0.,0.,1.));
#19787=DIRECTION('center_axis',(0.,1.,0.));
#19788=DIRECTION('ref_axis',(0.,0.,1.));
#19789=DIRECTION('center_axis',(0.,-1.,0.));
#19790=DIRECTION('ref_axis',(-1.22464679914735E-16,0.,1.));
#19791=DIRECTION('center_axis',(0.,1.,0.));
#19792=DIRECTION('ref_axis',(0.,0.,1.));
#19793=DIRECTION('center_axis',(0.,-1.,0.));
#19794=DIRECTION('ref_axis',(0.,0.,-1.));
#19795=DIRECTION('center_axis',(0.,-1.,0.));
#19796=DIRECTION('ref_axis',(0.,0.,-1.));
#19797=DIRECTION('center_axis',(0.,-1.,0.));
#19798=DIRECTION('ref_axis',(1.22464679914735E-16,0.,1.));
#19799=DIRECTION('center_axis',(0.,-1.,0.));
#19800=DIRECTION('ref_axis',(0.,0.,-1.));
#19801=DIRECTION('center_axis',(0.,-1.,0.));
#19802=DIRECTION('ref_axis',(0.,0.,-1.));
#19803=DIRECTION('',(0.,-1.,0.));
#19804=DIRECTION('center_axis',(0.,1.,0.));
#19805=DIRECTION('ref_axis',(0.,0.,1.));
#19806=DIRECTION('',(0.,1.,0.));
#19807=DIRECTION('center_axis',(0.,-1.,0.));
#19808=DIRECTION('ref_axis',(0.,0.,-1.));
#19809=DIRECTION('center_axis',(0.,1.,0.));
#19810=DIRECTION('ref_axis',(0.,0.,1.));
#19811=DIRECTION('',(0.,1.,0.));
#19812=DIRECTION('center_axis',(0.,1.,0.));
#19813=DIRECTION('ref_axis',(0.,0.,1.));
#19814=DIRECTION('',(0.,-1.,0.));
#19815=DIRECTION('center_axis',(0.,-1.,0.));
#19816=DIRECTION('ref_axis',(0.,0.,-1.));
#19817=DIRECTION('center_axis',(0.,1.,0.));
#19818=DIRECTION('ref_axis',(0.,0.,1.));
#19819=DIRECTION('',(0.,-1.,0.));
#19820=DIRECTION('center_axis',(0.,-1.,0.));
#19821=DIRECTION('ref_axis',(0.,0.,-1.));
#19822=DIRECTION('',(0.,1.,0.));
#19823=DIRECTION('center_axis',(0.,0.,-1.));
#19824=DIRECTION('ref_axis',(-1.,0.,0.));
#19825=DIRECTION('',(-1.,0.,0.));
#19826=DIRECTION('',(-1.,0.,0.));
#19827=DIRECTION('',(-1.,0.,0.));
#19828=DIRECTION('',(0.,1.,0.));
#19829=DIRECTION('',(1.,0.,0.));
#19830=DIRECTION('center_axis',(0.,0.,-1.));
#19831=DIRECTION('ref_axis',(-1.,0.,0.));
#19832=DIRECTION('',(-1.,0.,0.));
#19833=DIRECTION('',(1.,0.,0.));
#19834=DIRECTION('',(0.,-1.,0.));
#19835=DIRECTION('',(-1.,0.,0.));
#19836=DIRECTION('',(-1.,0.,0.));
#19837=DIRECTION('center_axis',(0.,1.,0.));
#19838=DIRECTION('ref_axis',(0.,0.,1.));
#19839=DIRECTION('center_axis',(0.,1.,0.));
#19840=DIRECTION('ref_axis',(0.,0.,1.));
#19841=DIRECTION('center_axis',(0.,1.,0.));
#19842=DIRECTION('ref_axis',(0.,0.,1.));
#19843=DIRECTION('center_axis',(0.,1.,0.));
#19844=DIRECTION('ref_axis',(0.,0.,1.));
#19845=DIRECTION('center_axis',(0.,1.,0.));
#19846=DIRECTION('ref_axis',(0.,0.,1.));
#19847=DIRECTION('center_axis',(0.,1.,0.));
#19848=DIRECTION('ref_axis',(-1.22464679914735E-16,0.,-1.));
#19849=DIRECTION('center_axis',(0.,-1.,0.));
#19850=DIRECTION('ref_axis',(0.,0.,-1.));
#19851=DIRECTION('center_axis',(1.,0.,0.));
#19852=DIRECTION('ref_axis',(0.,0.,-1.));
#19853=DIRECTION('',(0.,1.,0.));
#19854=DIRECTION('',(0.,0.,-1.));
#19855=DIRECTION('',(0.,1.,0.));
#19856=DIRECTION('',(0.,0.,1.));
#19857=DIRECTION('center_axis',(0.,0.,1.));
#19858=DIRECTION('ref_axis',(1.,0.,0.));
#19859=DIRECTION('',(0.,1.,0.));
#19860=DIRECTION('',(1.,0.,0.));
#19861=DIRECTION('',(-1.,0.,0.));
#19862=DIRECTION('',(0.,1.,0.));
#19863=DIRECTION('',(1.,0.,0.));
#19864=DIRECTION('',(0.,1.,0.));
#19865=DIRECTION('',(1.,0.,0.));
#19866=DIRECTION('center_axis',(0.,0.,-1.));
#19867=DIRECTION('ref_axis',(-1.,0.,0.));
#19868=DIRECTION('',(-1.,0.,0.));
#19869=DIRECTION('',(0.,-1.,0.));
#19870=DIRECTION('',(-1.,0.,0.));
#19871=DIRECTION('',(0.,1.,0.));
#19872=DIRECTION('',(-1.,0.,0.));
#19873=DIRECTION('',(0.,-1.,0.));
#19874=DIRECTION('',(1.,0.,0.));
#19875=DIRECTION('center_axis',(0.,1.,0.));
#19876=DIRECTION('ref_axis',(0.,0.,1.));
#19877=DIRECTION('center_axis',(0.,-1.,0.));
#19878=DIRECTION('ref_axis',(0.,0.,-1.));
#19879=DIRECTION('center_axis',(0.,-1.,0.));
#19880=DIRECTION('ref_axis',(0.,0.,1.));
#19881=DIRECTION('center_axis',(0.,1.,0.));
#19882=DIRECTION('ref_axis',(0.,0.,1.));
#19883=DIRECTION('center_axis',(0.,1.,0.));
#19884=DIRECTION('ref_axis',(0.,0.,1.));
#19885=DIRECTION('center_axis',(0.,-1.,0.));
#19886=DIRECTION('ref_axis',(0.,0.,1.));
#19887=DIRECTION('center_axis',(0.,1.,0.));
#19888=DIRECTION('ref_axis',(0.,0.,1.));
#19889=DIRECTION('center_axis',(0.,1.,0.));
#19890=DIRECTION('ref_axis',(0.,0.,1.));
#19891=DIRECTION('center_axis',(0.,1.,0.));
#19892=DIRECTION('ref_axis',(0.,0.,1.));
#19893=DIRECTION('center_axis',(0.,1.,0.));
#19894=DIRECTION('ref_axis',(0.,0.,1.));
#19895=DIRECTION('center_axis',(0.,-1.,0.));
#19896=DIRECTION('ref_axis',(0.,0.,-1.));
#19897=DIRECTION('center_axis',(0.,-1.,0.));
#19898=DIRECTION('ref_axis',(0.,0.,-1.));
#19899=DIRECTION('center_axis',(0.,-1.,0.));
#19900=DIRECTION('ref_axis',(0.,0.,-1.));
#19901=DIRECTION('center_axis',(-1.,0.,0.));
#19902=DIRECTION('ref_axis',(0.,0.,1.));
#19903=DIRECTION('',(0.,1.,0.));
#19904=DIRECTION('',(0.,0.,1.));
#19905=DIRECTION('',(0.,1.,0.));
#19906=DIRECTION('',(0.,0.,-1.));
#19907=DIRECTION('center_axis',(0.,0.,-1.));
#19908=DIRECTION('ref_axis',(-1.,0.,0.));
#19909=DIRECTION('',(0.,1.,0.));
#19910=DIRECTION('',(-1.,0.,0.));
#19911=DIRECTION('',(1.,0.,0.));
#19912=DIRECTION('',(0.,1.,0.));
#19913=DIRECTION('',(-1.,0.,0.));
#19914=DIRECTION('',(0.,1.,0.));
#19915=DIRECTION('',(-1.,0.,0.));
#19916=DIRECTION('center_axis',(0.,0.,1.));
#19917=DIRECTION('ref_axis',(1.,0.,0.));
#19918=DIRECTION('',(1.,0.,0.));
#19919=DIRECTION('',(0.,-1.,0.));
#19920=DIRECTION('',(1.,0.,0.));
#19921=DIRECTION('',(0.,1.,0.));
#19922=DIRECTION('',(1.,0.,0.));
#19923=DIRECTION('',(0.,-1.,0.));
#19924=DIRECTION('',(-1.,0.,0.));
#19925=DIRECTION('center_axis',(0.,1.,0.));
#19926=DIRECTION('ref_axis',(0.,0.,1.));
#19927=DIRECTION('center_axis',(0.,-1.,0.));
#19928=DIRECTION('ref_axis',(0.,0.,-1.));
#19929=DIRECTION('center_axis',(0.,-1.,0.));
#19930=DIRECTION('ref_axis',(0.,0.,1.));
#19931=DIRECTION('center_axis',(0.,1.,0.));
#19932=DIRECTION('ref_axis',(0.,0.,1.));
#19933=DIRECTION('center_axis',(0.,1.,0.));
#19934=DIRECTION('ref_axis',(0.,0.,1.));
#19935=DIRECTION('center_axis',(0.,-1.,0.));
#19936=DIRECTION('ref_axis',(0.,0.,1.));
#19937=DIRECTION('center_axis',(0.,1.,0.));
#19938=DIRECTION('ref_axis',(0.,0.,1.));
#19939=DIRECTION('center_axis',(0.,1.,0.));
#19940=DIRECTION('ref_axis',(0.,0.,1.));
#19941=DIRECTION('center_axis',(0.,1.,0.));
#19942=DIRECTION('ref_axis',(0.,0.,1.));
#19943=DIRECTION('center_axis',(0.,1.,0.));
#19944=DIRECTION('ref_axis',(0.,0.,1.));
#19945=DIRECTION('center_axis',(0.,-1.,0.));
#19946=DIRECTION('ref_axis',(0.,0.,-1.));
#19947=DIRECTION('center_axis',(0.,-1.,0.));
#19948=DIRECTION('ref_axis',(0.,0.,-1.));
#19949=DIRECTION('center_axis',(0.,-1.,0.));
#19950=DIRECTION('ref_axis',(0.,0.,-1.));
#24600=CARTESIAN_POINT('',(0.,0.,0.));
#24601=CARTESIAN_POINT('Origin',(0.,27.,0.));
#24602=CARTESIAN_POINT('',(-22.477766792989,27.,1.));
#24603=CARTESIAN_POINT('',(22.477766792989,27.,1.));
#24604=CARTESIAN_POINT('Origin',(0.,27.,0.));
#24605=CARTESIAN_POINT('',(22.477766792989,34.,1.));
#24606=CARTESIAN_POINT('',(22.477766792989,27.,1.));
#24607=CARTESIAN_POINT('',(-22.477766792989,34.,1.));
#24608=CARTESIAN_POINT('Origin',(0.,34.,0.));
#24609=CARTESIAN_POINT('',(-22.477766792989,27.,1.));
#24610=CARTESIAN_POINT('Origin',(0.,34.,0.));
#24611=CARTESIAN_POINT('',(24.9799919935936,5.,1.));
#24612=CARTESIAN_POINT('',(-24.9799919935936,5.,1.));
#24613=CARTESIAN_POINT('Origin',(0.,5.,0.));
#24614=CARTESIAN_POINT('',(24.9799919935936,27.,1.));
#24615=CARTESIAN_POINT('',(24.9799919935936,34.,1.));
#24616=CARTESIAN_POINT('',(-24.9799919935936,27.,1.));
#24617=CARTESIAN_POINT('Origin',(0.,27.,0.));
#24618=CARTESIAN_POINT('',(-24.9799919935936,34.,1.));
#24619=CARTESIAN_POINT('Origin',(-26.2146741366494,0.,1.));
#24620=CARTESIAN_POINT('',(22.477766792989,5.,1.));
#24621=CARTESIAN_POINT('',(-26.2146741366494,5.,1.));
#24622=CARTESIAN_POINT('',(22.477766792989,0.,1.));
#24623=CARTESIAN_POINT('',(22.477766792989,5.,1.));
#24624=CARTESIAN_POINT('',(10.4522724801834,0.,1.));
#24625=CARTESIAN_POINT('',(-26.2146741366494,0.,1.));
#24626=CARTESIAN_POINT('',(10.4522724801834,34.,1.));
#24627=CARTESIAN_POINT('',(10.4522724801834,34.,1.));
#24628=CARTESIAN_POINT('',(-26.2146741366494,34.,1.));
#24629=CARTESIAN_POINT('',(-26.2146741366494,27.,1.));
#24630=CARTESIAN_POINT('Origin',(-26.2146741366494,0.,1.));
#24631=CARTESIAN_POINT('',(-22.477766792989,5.,1.));
#24632=CARTESIAN_POINT('',(-26.2146741366494,5.,1.));
#24633=CARTESIAN_POINT('',(-26.2146741366494,27.,1.));
#24634=CARTESIAN_POINT('',(-10.4522724801834,34.,1.));
#24635=CARTESIAN_POINT('',(-26.2146741366494,34.,1.));
#24636=CARTESIAN_POINT('',(-10.4522724801834,0.,1.));
#24637=CARTESIAN_POINT('',(-10.4522724801834,34.,1.));
#24638=CARTESIAN_POINT('',(-22.477766792989,0.,1.));
#24639=CARTESIAN_POINT('',(-26.2146741366494,0.,1.));
#24640=CARTESIAN_POINT('',(-22.477766792989,5.,1.));
#24641=CARTESIAN_POINT('Origin',(0.,0.,0.));
#24642=CARTESIAN_POINT('Origin',(0.,0.,0.));
#24643=CARTESIAN_POINT('Origin',(0.,0.,0.));
#24644=CARTESIAN_POINT('Origin',(0.,34.,0.));
#24645=CARTESIAN_POINT('Origin',(0.,34.,0.));
#24646=CARTESIAN_POINT('Origin',(0.,34.,0.));
#24647=CARTESIAN_POINT('Origin',(0.,27.,0.));
#24648=CARTESIAN_POINT('Origin',(0.,5.,0.));
#24649=CARTESIAN_POINT('Origin',(0.,5.,0.));
#24650=CARTESIAN_POINT('Origin',(0.,5.,0.));
#24651=CARTESIAN_POINT('Origin',(0.,5.,0.));
#24652=CARTESIAN_POINT('',(-22.477766792989,5.,-1.));
#24653=CARTESIAN_POINT('',(22.477766792989,5.,-1.));
#24654=CARTESIAN_POINT('Origin',(0.,5.,0.));
#24655=CARTESIAN_POINT('',(22.477766792989,0.,-1.));
#24656=CARTESIAN_POINT('',(22.477766792989,5.,-1.));
#24657=CARTESIAN_POINT('',(-22.477766792989,0.,-1.));
#24658=CARTESIAN_POINT('Origin',(0.,0.,0.));
#24659=CARTESIAN_POINT('',(-22.477766792989,5.,-1.));
#24660=CARTESIAN_POINT('Origin',(0.,34.,0.));
#24661=CARTESIAN_POINT('',(10.4522724801834,34.,-1.));
#24662=CARTESIAN_POINT('',(-10.4522724801834,34.,-1.));
#24663=CARTESIAN_POINT('Origin',(0.,34.,0.));
#24664=CARTESIAN_POINT('',(-10.4522724801834,0.,-1.));
#24665=CARTESIAN_POINT('',(-10.4522724801834,34.,-1.));
#24666=CARTESIAN_POINT('',(10.4522724801834,0.,-1.));
#24667=CARTESIAN_POINT('Origin',(0.,0.,0.));
#24668=CARTESIAN_POINT('',(10.4522724801834,34.,-1.));
#24669=CARTESIAN_POINT('Origin',(0.,34.,0.));
#24670=CARTESIAN_POINT('',(24.9799919935936,27.,-1.));
#24671=CARTESIAN_POINT('',(-24.9799919935936,27.,-1.));
#24672=CARTESIAN_POINT('Origin',(0.,27.,0.));
#24673=CARTESIAN_POINT('',(24.9799919935936,5.,-1.));
#24674=CARTESIAN_POINT('',(24.9799919935936,34.,-1.));
#24675=CARTESIAN_POINT('',(-24.9799919935936,5.,-1.));
#24676=CARTESIAN_POINT('Origin',(0.,5.,0.));
#24677=CARTESIAN_POINT('',(-24.9799919935936,34.,-1.));
#24678=CARTESIAN_POINT('Origin',(-26.2146741366494,0.,-1.));
#24679=CARTESIAN_POINT('',(-26.2146741366494,5.,-1.));
#24680=CARTESIAN_POINT('',(-26.2146741366494,0.,-1.));
#24681=CARTESIAN_POINT('',(-22.477766792989,34.,-1.));
#24682=CARTESIAN_POINT('',(-26.2146741366494,34.,-1.));
#24683=CARTESIAN_POINT('',(-22.477766792989,27.,-1.));
#24684=CARTESIAN_POINT('',(-22.477766792989,27.,-1.));
#24685=CARTESIAN_POINT('',(-26.2146741366494,27.,-1.));
#24686=CARTESIAN_POINT('Origin',(-26.2146741366494,0.,-1.));
#24687=CARTESIAN_POINT('',(-26.2146741366494,5.,-1.));
#24688=CARTESIAN_POINT('',(22.477766792989,27.,-1.));
#24689=CARTESIAN_POINT('',(-26.2146741366494,27.,-1.));
#24690=CARTESIAN_POINT('',(22.477766792989,34.,-1.));
#24691=CARTESIAN_POINT('',(22.477766792989,27.,-1.));
#24692=CARTESIAN_POINT('',(-26.2146741366494,34.,-1.));
#24693=CARTESIAN_POINT('',(-26.2146741366494,0.,-1.));
#24694=CARTESIAN_POINT('Origin',(0.,0.,0.));
#24695=CARTESIAN_POINT('Origin',(0.,34.,0.));
#24696=CARTESIAN_POINT('Origin',(0.,34.,0.));
#24697=CARTESIAN_POINT('Origin',(0.,27.,0.));
#24698=CARTESIAN_POINT('Origin',(0.,27.,0.));
#24699=CARTESIAN_POINT('Origin',(0.,27.,0.));
#24700=CARTESIAN_POINT('Origin',(0.,5.,0.));
#24701=CARTESIAN_POINT('Origin',(24.9799919935936,0.,-1.));
#24702=CARTESIAN_POINT('',(24.9799919935936,5.,1.));
#24703=CARTESIAN_POINT('',(24.9799919935936,27.,1.));
#24704=CARTESIAN_POINT('',(24.9799919935936,0.,1.));
#24705=CARTESIAN_POINT('',(24.9799919935936,5.,-1.));
#24706=CARTESIAN_POINT('',(24.9799919935936,5.,-1.));
#24707=CARTESIAN_POINT('',(24.9799919935936,27.,-1.));
#24708=CARTESIAN_POINT('',(24.9799919935936,0.,-1.));
#24709=CARTESIAN_POINT('',(24.9799919935936,27.,-1.));
#24710=CARTESIAN_POINT('Origin',(10.4522724801834,0.,1.));
#24711=CARTESIAN_POINT('',(22.477766792989,0.,1.));
#24712=CARTESIAN_POINT('',(22.477766792989,5.,1.));
#24713=CARTESIAN_POINT('',(22.477766792989,5.,1.));
#24714=CARTESIAN_POINT('',(10.4522724801834,5.,1.));
#24715=CARTESIAN_POINT('',(22.477766792989,27.,1.));
#24716=CARTESIAN_POINT('',(10.4522724801834,27.,1.));
#24717=CARTESIAN_POINT('',(22.477766792989,34.,1.));
#24718=CARTESIAN_POINT('',(22.477766792989,27.,1.));
#24719=CARTESIAN_POINT('',(10.4522724801834,34.,1.));
#24720=CARTESIAN_POINT('',(10.4522724801834,34.,1.));
#24721=CARTESIAN_POINT('',(10.4522724801834,0.,1.));
#24722=CARTESIAN_POINT('',(10.4522724801834,0.,1.));
#24723=CARTESIAN_POINT('',(10.4522724801834,0.,1.));
#24724=CARTESIAN_POINT('Origin',(10.4522724801834,0.,-1.));
#24725=CARTESIAN_POINT('',(22.477766792989,5.,-1.));
#24726=CARTESIAN_POINT('',(10.4522724801834,5.,-1.));
#24727=CARTESIAN_POINT('',(22.477766792989,0.,-1.));
#24728=CARTESIAN_POINT('',(22.477766792989,5.,-1.));
#24729=CARTESIAN_POINT('',(10.4522724801834,0.,-1.));
#24730=CARTESIAN_POINT('',(10.4522724801834,0.,-1.));
#24731=CARTESIAN_POINT('',(10.4522724801834,34.,-1.));
#24732=CARTESIAN_POINT('',(10.4522724801834,0.,-1.));
#24733=CARTESIAN_POINT('',(22.477766792989,34.,-1.));
#24734=CARTESIAN_POINT('',(10.4522724801834,34.,-1.));
#24735=CARTESIAN_POINT('',(22.477766792989,27.,-1.));
#24736=CARTESIAN_POINT('',(22.477766792989,27.,-1.));
#24737=CARTESIAN_POINT('',(10.4522724801834,27.,-1.));
#24738=CARTESIAN_POINT('Origin',(-3.46944695195361E-15,0.,2.16840434497101E-16));
#24739=CARTESIAN_POINT('Origin',(0.,0.,0.));
#24740=CARTESIAN_POINT('Origin',(-3.46944695195361E-15,0.,2.16840434497101E-16));
#24741=CARTESIAN_POINT('Origin',(-3.46944695195361E-15,34.,2.16840434497101E-16));
#24742=CARTESIAN_POINT('Origin',(0.,34.,0.));
#24743=CARTESIAN_POINT('Origin',(-3.46944695195361E-15,34.,2.16840434497101E-16));
#24744=CARTESIAN_POINT('Origin',(-3.46944695195361E-15,0.,2.16840434497101E-16));
#24745=CARTESIAN_POINT('Origin',(0.,27.,0.));
#24746=CARTESIAN_POINT('Origin',(0.,27.,0.));
#24747=CARTESIAN_POINT('Origin',(0.,27.,0.));
#24748=CARTESIAN_POINT('Origin',(0.,5.,0.));
#24749=CARTESIAN_POINT('Origin',(0.,5.,0.));
#24750=CARTESIAN_POINT('Origin',(0.,5.,0.));
#24751=CARTESIAN_POINT('Origin',(-24.9799919935936,0.,-1.));
#24752=CARTESIAN_POINT('',(-24.9799919935936,5.,-1.));
#24753=CARTESIAN_POINT('',(-24.9799919935936,27.,-1.));
#24754=CARTESIAN_POINT('',(-24.9799919935936,0.,-1.));
#24755=CARTESIAN_POINT('',(-24.9799919935936,5.,1.));
#24756=CARTESIAN_POINT('',(-24.9799919935936,5.,-1.));
#24757=CARTESIAN_POINT('',(-24.9799919935936,27.,1.));
#24758=CARTESIAN_POINT('',(-24.9799919935936,0.,1.));
#24759=CARTESIAN_POINT('',(-24.9799919935936,27.,-1.));
#24760=CARTESIAN_POINT('Origin',(-24.9799919935936,0.,-1.));
#24761=CARTESIAN_POINT('',(-22.477766792989,0.,-1.));
#24762=CARTESIAN_POINT('',(-22.477766792989,5.,-1.));
#24763=CARTESIAN_POINT('',(-22.477766792989,5.,-1.));
#24764=CARTESIAN_POINT('',(-24.9799919935936,5.,-1.));
#24765=CARTESIAN_POINT('',(-22.477766792989,27.,-1.));
#24766=CARTESIAN_POINT('',(-24.9799919935936,27.,-1.));
#24767=CARTESIAN_POINT('',(-22.477766792989,34.,-1.));
#24768=CARTESIAN_POINT('',(-22.477766792989,27.,-1.));
#24769=CARTESIAN_POINT('',(-10.4522724801834,34.,-1.));
#24770=CARTESIAN_POINT('',(-24.9799919935936,34.,-1.));
#24771=CARTESIAN_POINT('',(-10.4522724801834,0.,-1.));
#24772=CARTESIAN_POINT('',(-10.4522724801834,0.,-1.));
#24773=CARTESIAN_POINT('',(-24.9799919935936,0.,-1.));
#24774=CARTESIAN_POINT('Origin',(-24.9799919935936,0.,1.));
#24775=CARTESIAN_POINT('',(-22.477766792989,5.,1.));
#24776=CARTESIAN_POINT('',(-24.9799919935936,5.,1.));
#24777=CARTESIAN_POINT('',(-22.477766792989,0.,1.));
#24778=CARTESIAN_POINT('',(-22.477766792989,5.,1.));
#24779=CARTESIAN_POINT('',(-10.4522724801834,0.,0.999999999999992));
#24780=CARTESIAN_POINT('',(-24.9799919935936,0.,1.));
#24781=CARTESIAN_POINT('',(-10.4522724801834,34.,0.999999999999992));
#24782=CARTESIAN_POINT('',(-10.4522724801834,0.,0.999999999999992));
#24783=CARTESIAN_POINT('',(-22.477766792989,34.,1.));
#24784=CARTESIAN_POINT('',(-24.9799919935936,34.,1.));
#24785=CARTESIAN_POINT('',(-22.477766792989,27.,1.));
#24786=CARTESIAN_POINT('',(-22.477766792989,27.,1.));
#24787=CARTESIAN_POINT('',(-24.9799919935936,27.,1.));
#24788=CARTESIAN_POINT('Origin',(-3.46944695195361E-15,0.,2.16840434497101E-16));
#24789=CARTESIAN_POINT('Origin',(0.,0.,0.));
#24790=CARTESIAN_POINT('Origin',(-3.46944695195361E-15,0.,2.16840434497101E-16));
#24791=CARTESIAN_POINT('Origin',(-3.46944695195361E-15,34.,2.16840434497101E-16));
#24792=CARTESIAN_POINT('Origin',(0.,34.,0.));
#24793=CARTESIAN_POINT('Origin',(-3.46944695195361E-15,34.,2.16840434497101E-16));
#24794=CARTESIAN_POINT('Origin',(-3.46944695195361E-15,0.,2.16840434497101E-16));
#24795=CARTESIAN_POINT('Origin',(0.,27.,0.));
#24796=CARTESIAN_POINT('Origin',(0.,27.,0.));
#24797=CARTESIAN_POINT('Origin',(0.,27.,0.));
#24798=CARTESIAN_POINT('Origin',(0.,5.,0.));
#24799=CARTESIAN_POINT('Origin',(0.,5.,0.));
#24800=CARTESIAN_POINT('Origin',(0.,5.,0.));
#38605=UNCERTAINTY_MEASURE_WITH_UNIT(LENGTH_MEASURE(0.01),#38636,
'DISTANCE_ACCURACY_VALUE',
'Maximum model space distance between geometric entities at asserted c
onnectivities');
#38619=UNCERTAINTY_MEASURE_WITH_UNIT(LENGTH_MEASURE(0.01),#38636,
'DISTANCE_ACCURACY_VALUE',
'Maximum model space distance between geometric entities at asserted c
onnectivities');
#38621=(
GEOMETRIC_REPRESENTATION_CONTEXT(3)
GLOBAL_UNCERTAINTY_ASSIGNED_CONTEXT((#38605))
GLOBAL_UNIT_ASSIGNED_CONTEXT((#38636,#38638,#38639))
REPRESENTATION_CONTEXT('','3D')
);
#38635=(
GEOMETRIC_REPRESENTATION_CONTEXT(3)
GLOBAL_UNCERTAINTY_ASSIGNED_CONTEXT((#38619))
GLOBAL_UNIT_ASSIGNED_CONTEXT((#38636,#38638,#38639))
REPRESENTATION_CONTEXT('','3D')
);
#38636=(
LENGTH_UNIT()
NAMED_UNIT(*)
SI_UNIT(.MILLI.,.METRE.)
);
#38638=(
NAMED_UNIT(*)
PLANE_ANGLE_UNIT()
SI_UNIT($,.RADIAN.)
);
#38639=(
NAMED_UNIT(*)
SI_UNIT($,.STERADIAN.)
SOLID_ANGLE_UNIT()
);
#38641=SHAPE_DEFINITION_REPRESENTATION(#38656,#38685);
#38656=PRODUCT_DEFINITION_SHAPE('',$,#38701);
#38685=SHAPE_REPRESENTATION('',(#17788),#38621);
#38699=PRODUCT_DEFINITION_CONTEXT('part definition',#38746,'design');
#38701=PRODUCT_DEFINITION('Magnetic Base','Magnetic Base',#38716,#38699);
#38716=PRODUCT_DEFINITION_FORMATION('',$,#38749);
#38746=APPLICATION_CONTEXT(
'Core Data for Automotive Mechanical Design Process');
#38747=PRODUCT_CONTEXT('part definition',#38746,'mechanical');
#38749=PRODUCT('Magnetic Base','Magnetic Base',$,(#38747));
#38764=PRESENTATION_STYLE_ASSIGNMENT((#38771));
#38771=SURFACE_STYLE_USAGE(.BOTH.,#38778);
#38778=SURFACE_SIDE_STYLE('',(#38785));
#38785=SURFACE_STYLE_FILL_AREA(#38792);
#38792=FILL_AREA_STYLE('Opaque(20,51,87)',(#38799));
#38799=FILL_AREA_STYLE_COLOUR('Opaque(20,51,87)',#38806);
#38806=COLOUR_RGB('Opaque(20,51,87)',0.0784313725490196,0.2,0.341176470588235);
ENDSEC;
END-ISO-10303-21;
